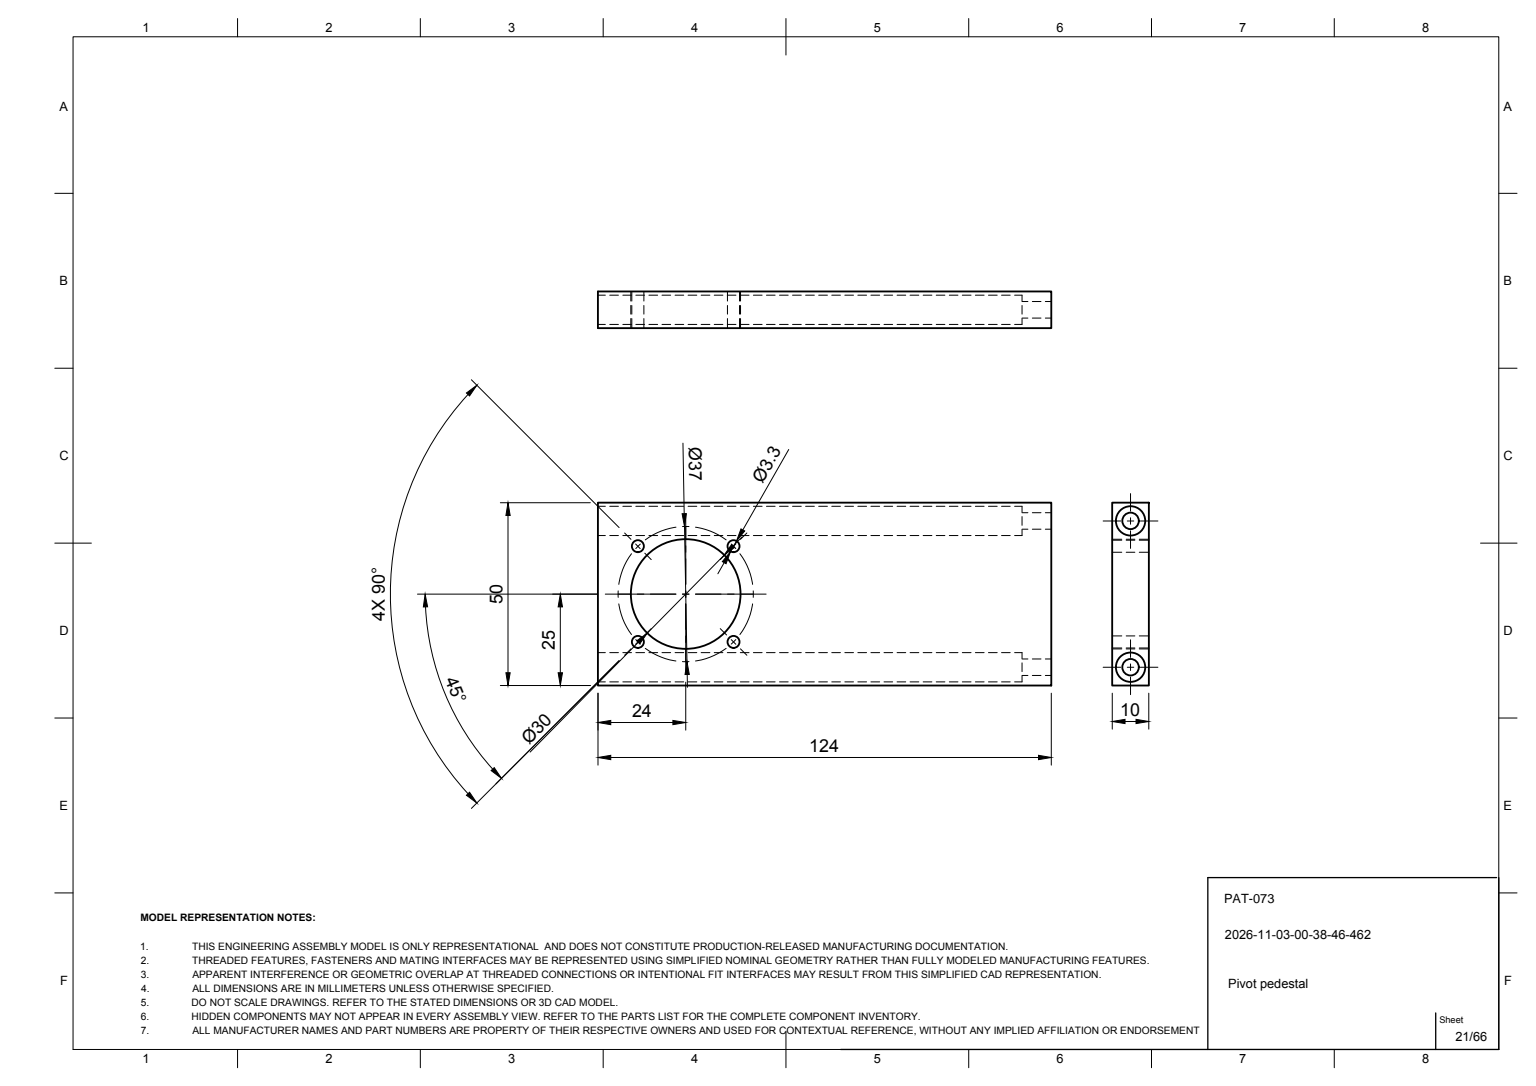
ISO-10303-21;
HEADER;
/* Generated by software containing ST-Developer
 * from STEP Tools, Inc. (www.steptools.com) 
 */

FILE_DESCRIPTION(
/* description */ ('Manual piston pump'),
/* implementation_level */ '2;1');

FILE_NAME(
/* name */ 'Pivot pedestal.step',
/* time_stamp */ '2026-11-02T16:54:23-08:00',
/* author */ (''),
/* organization */ (''),
/* preprocessor_version */ 'ST-DEVELOPER v20.2',
/* originating_system */ 'Autodesk Translation Framework v15.17.0.0',
/* authorisation */ '');

FILE_SCHEMA (('AUTOMOTIVE_DESIGN { 1 0 10303 214 3 1 1 }'));
ENDSEC;

DATA;
#10=MECHANICAL_DESIGN_GEOMETRIC_PRESENTATION_REPRESENTATION('',(#707),#19043);
#581=SHAPE_REPRESENTATION_RELATIONSHIP('SRR','None',#19327,#644);
#644=ADVANCED_BREP_SHAPE_REPRESENTATION('',(#778),#18994);
#707=STYLED_ITEM('',(#19661),#778);
#778=MANIFOLD_SOLID_BREP('Body1',#9492);
#901=FACE_BOUND('',#2123,.T.);
#902=FACE_BOUND('',#2127,.T.);
#903=FACE_BOUND('',#2131,.T.);
#904=FACE_BOUND('',#2132,.T.);
#905=FACE_BOUND('',#2135,.T.);
#906=FACE_BOUND('',#2136,.T.);
#907=FACE_BOUND('',#2139,.T.);
#908=FACE_BOUND('',#2140,.T.);
#909=FACE_BOUND('',#2141,.T.);
#910=FACE_BOUND('',#2142,.T.);
#911=FACE_BOUND('',#2143,.T.);
#912=FACE_BOUND('',#2145,.T.);
#913=FACE_BOUND('',#2146,.T.);
#914=FACE_BOUND('',#2147,.T.);
#915=FACE_BOUND('',#2148,.T.);
#916=FACE_BOUND('',#2149,.T.);
#1155=CYLINDRICAL_SURFACE('',#10580,0.164999999999999);
#1156=CYLINDRICAL_SURFACE('',#10583,0.164999999999999);
#1157=CYLINDRICAL_SURFACE('',#10586,0.164999999999999);
#1158=CYLINDRICAL_SURFACE('',#10589,0.164999999999999);
#1159=CYLINDRICAL_SURFACE('',#10592,0.4);
#1160=CYLINDRICAL_SURFACE('',#10597,0.225);
#1161=CYLINDRICAL_SURFACE('',#10599,0.4);
#1162=CYLINDRICAL_SURFACE('',#10604,0.225);
#1163=CYLINDRICAL_SURFACE('',#10606,1.5);
#1468=FACE_OUTER_BOUND('',#2117,.T.);
#1469=FACE_OUTER_BOUND('',#2118,.T.);
#1470=FACE_OUTER_BOUND('',#2119,.T.);
#1471=FACE_OUTER_BOUND('',#2120,.T.);
#1472=FACE_OUTER_BOUND('',#2121,.T.);
#1473=FACE_OUTER_BOUND('',#2122,.T.);
#1474=FACE_OUTER_BOUND('',#2124,.T.);
#1475=FACE_OUTER_BOUND('',#2125,.T.);
#1476=FACE_OUTER_BOUND('',#2126,.T.);
#1477=FACE_OUTER_BOUND('',#2128,.T.);
#1478=FACE_OUTER_BOUND('',#2129,.T.);
#1479=FACE_OUTER_BOUND('',#2130,.T.);
#1480=FACE_OUTER_BOUND('',#2133,.T.);
#1481=FACE_OUTER_BOUND('',#2134,.T.);
#1482=FACE_OUTER_BOUND('',#2137,.T.);
#1483=FACE_OUTER_BOUND('',#2138,.T.);
#1484=FACE_OUTER_BOUND('',#2144,.T.);
#2117=EDGE_LOOP('',(#6985,#6986,#6987,#6988));
#2118=EDGE_LOOP('',(#6989,#6990,#6991,#6992));
#2119=EDGE_LOOP('',(#6993,#6994,#6995,#6996));
#2120=EDGE_LOOP('',(#6997,#6998,#6999,#7000));
#2121=EDGE_LOOP('',(#7001,#7002,#7003,#7004));
#2122=EDGE_LOOP('',(#7005));
#2123=EDGE_LOOP('',(#7006));
#2124=EDGE_LOOP('',(#7007,#7008,#7009,#7010));
#2125=EDGE_LOOP('',(#7011,#7012,#7013,#7014));
#2126=EDGE_LOOP('',(#7015));
#2127=EDGE_LOOP('',(#7016));
#2128=EDGE_LOOP('',(#7017,#7018,#7019,#7020));
#2129=EDGE_LOOP('',(#7021,#7022,#7023,#7024));
#2130=EDGE_LOOP('',(#7025,#7026,#7027,#7028));
#2131=EDGE_LOOP('',(#7029));
#2132=EDGE_LOOP('',(#7030));
#2133=EDGE_LOOP('',(#7031,#7032,#7033,#7034));
#2134=EDGE_LOOP('',(#7035,#7036,#7037,#7038));
#2135=EDGE_LOOP('',(#7039));
#2136=EDGE_LOOP('',(#7040));
#2137=EDGE_LOOP('',(#7041,#7042,#7043,#7044));
#2138=EDGE_LOOP('',(#7045,#7046,#7047,#7048));
#2139=EDGE_LOOP('',(#7049));
#2140=EDGE_LOOP('',(#7050));
#2141=EDGE_LOOP('',(#7051));
#2142=EDGE_LOOP('',(#7052));
#2143=EDGE_LOOP('',(#7053));
#2144=EDGE_LOOP('',(#7054,#7055,#7056,#7057));
#2145=EDGE_LOOP('',(#7058));
#2146=EDGE_LOOP('',(#7059));
#2147=EDGE_LOOP('',(#7060));
#2148=EDGE_LOOP('',(#7061));
#2149=EDGE_LOOP('',(#7062));
#2802=CIRCLE('',#10581,0.164999999999999);
#2803=CIRCLE('',#10582,0.164999999999999);
#2804=CIRCLE('',#10584,0.164999999999999);
#2805=CIRCLE('',#10585,0.164999999999999);
#2806=CIRCLE('',#10587,0.164999999999999);
#2807=CIRCLE('',#10588,0.164999999999999);
#2808=CIRCLE('',#10590,0.164999999999999);
#2809=CIRCLE('',#10591,0.164999999999999);
#2810=CIRCLE('',#10593,0.4);
#2811=CIRCLE('',#10594,0.4);
#2812=CIRCLE('',#10596,0.225);
#2813=CIRCLE('',#10598,0.225);
#2814=CIRCLE('',#10600,0.4);
#2815=CIRCLE('',#10601,0.4);
#2816=CIRCLE('',#10603,0.225);
#2817=CIRCLE('',#10605,0.225);
#2818=CIRCLE('',#10607,1.5);
#2819=CIRCLE('',#10608,1.5);
#3349=LINE('',#15470,#3953);
#3350=LINE('',#15476,#3954);
#3351=LINE('',#15482,#3955);
#3352=LINE('',#15488,#3956);
#3353=LINE('',#15494,#3957);
#3354=LINE('',#15502,#3958);
#3355=LINE('',#15507,#3959);
#3356=LINE('',#15515,#3960);
#3357=LINE('',#15520,#3961);
#3358=LINE('',#15525,#3962);
#3359=LINE('',#15527,#3963);
#3360=LINE('',#15529,#3964);
#3361=LINE('',#15530,#3965);
#3362=LINE('',#15533,#3966);
#3363=LINE('',#15535,#3967);
#3364=LINE('',#15536,#3968);
#3365=LINE('',#15539,#3969);
#3366=LINE('',#15541,#3970);
#3367=LINE('',#15542,#3971);
#3368=LINE('',#15544,#3972);
#3369=LINE('',#15545,#3973);
#3953=VECTOR('',#12375,0.164999999999999);
#3954=VECTOR('',#12382,0.164999999999999);
#3955=VECTOR('',#12389,0.164999999999999);
#3956=VECTOR('',#12396,0.164999999999999);
#3957=VECTOR('',#12403,0.4);
#3958=VECTOR('',#12414,0.225);
#3959=VECTOR('',#12419,0.4);
#3960=VECTOR('',#12430,0.225);
#3961=VECTOR('',#12435,1.5);
#3962=VECTOR('',#12440,1.);
#3963=VECTOR('',#12441,1.);
#3964=VECTOR('',#12442,1.);
#3965=VECTOR('',#12443,1.);
#3966=VECTOR('',#12446,1.);
#3967=VECTOR('',#12447,1.);
#3968=VECTOR('',#12448,1.);
#3969=VECTOR('',#12451,1.);
#3970=VECTOR('',#12452,1.);
#3971=VECTOR('',#12453,1.);
#3972=VECTOR('',#12456,1.);
#3973=VECTOR('',#12457,1.);
#4589=VERTEX_POINT('',#15467);
#4590=VERTEX_POINT('',#15469);
#4591=VERTEX_POINT('',#15473);
#4592=VERTEX_POINT('',#15475);
#4593=VERTEX_POINT('',#15479);
#4594=VERTEX_POINT('',#15481);
#4595=VERTEX_POINT('',#15485);
#4596=VERTEX_POINT('',#15487);
#4597=VERTEX_POINT('',#15491);
#4598=VERTEX_POINT('',#15493);
#4599=VERTEX_POINT('',#15497);
#4600=VERTEX_POINT('',#15500);
#4601=VERTEX_POINT('',#15504);
#4602=VERTEX_POINT('',#15506);
#4603=VERTEX_POINT('',#15510);
#4604=VERTEX_POINT('',#15513);
#4605=VERTEX_POINT('',#15517);
#4606=VERTEX_POINT('',#15519);
#4607=VERTEX_POINT('',#15523);
#4608=VERTEX_POINT('',#15524);
#4609=VERTEX_POINT('',#15526);
#4610=VERTEX_POINT('',#15528);
#4611=VERTEX_POINT('',#15532);
#4612=VERTEX_POINT('',#15534);
#4613=VERTEX_POINT('',#15538);
#4614=VERTEX_POINT('',#15540);
#5479=EDGE_CURVE('',#4589,#4589,#2802,.T.);
#5480=EDGE_CURVE('',#4589,#4590,#3349,.T.);
#5481=EDGE_CURVE('',#4590,#4590,#2803,.T.);
#5482=EDGE_CURVE('',#4591,#4591,#2804,.T.);
#5483=EDGE_CURVE('',#4591,#4592,#3350,.T.);
#5484=EDGE_CURVE('',#4592,#4592,#2805,.T.);
#5485=EDGE_CURVE('',#4593,#4593,#2806,.T.);
#5486=EDGE_CURVE('',#4593,#4594,#3351,.T.);
#5487=EDGE_CURVE('',#4594,#4594,#2807,.T.);
#5488=EDGE_CURVE('',#4595,#4595,#2808,.T.);
#5489=EDGE_CURVE('',#4595,#4596,#3352,.T.);
#5490=EDGE_CURVE('',#4596,#4596,#2809,.T.);
#5491=EDGE_CURVE('',#4597,#4597,#2810,.T.);
#5492=EDGE_CURVE('',#4597,#4598,#3353,.T.);
#5493=EDGE_CURVE('',#4598,#4598,#2811,.T.);
#5494=EDGE_CURVE('',#4599,#4599,#2812,.T.);
#5495=EDGE_CURVE('',#4600,#4600,#2813,.T.);
#5496=EDGE_CURVE('',#4600,#4599,#3354,.T.);
#5497=EDGE_CURVE('',#4601,#4601,#2814,.T.);
#5498=EDGE_CURVE('',#4601,#4602,#3355,.T.);
#5499=EDGE_CURVE('',#4602,#4602,#2815,.T.);
#5500=EDGE_CURVE('',#4603,#4603,#2816,.T.);
#5501=EDGE_CURVE('',#4604,#4604,#2817,.T.);
#5502=EDGE_CURVE('',#4604,#4603,#3356,.T.);
#5503=EDGE_CURVE('',#4605,#4605,#2818,.T.);
#5504=EDGE_CURVE('',#4605,#4606,#3357,.T.);
#5505=EDGE_CURVE('',#4606,#4606,#2819,.T.);
#5506=EDGE_CURVE('',#4607,#4608,#3358,.T.);
#5507=EDGE_CURVE('',#4608,#4609,#3359,.T.);
#5508=EDGE_CURVE('',#4610,#4609,#3360,.T.);
#5509=EDGE_CURVE('',#4607,#4610,#3361,.T.);
#5510=EDGE_CURVE('',#4611,#4607,#3362,.T.);
#5511=EDGE_CURVE('',#4612,#4610,#3363,.T.);
#5512=EDGE_CURVE('',#4611,#4612,#3364,.T.);
#5513=EDGE_CURVE('',#4613,#4611,#3365,.T.);
#5514=EDGE_CURVE('',#4614,#4612,#3366,.T.);
#5515=EDGE_CURVE('',#4613,#4614,#3367,.T.);
#5516=EDGE_CURVE('',#4608,#4613,#3368,.T.);
#5517=EDGE_CURVE('',#4609,#4614,#3369,.T.);
#6985=ORIENTED_EDGE('',*,*,#5479,.F.);
#6986=ORIENTED_EDGE('',*,*,#5480,.T.);
#6987=ORIENTED_EDGE('',*,*,#5481,.F.);
#6988=ORIENTED_EDGE('',*,*,#5480,.F.);
#6989=ORIENTED_EDGE('',*,*,#5482,.F.);
#6990=ORIENTED_EDGE('',*,*,#5483,.T.);
#6991=ORIENTED_EDGE('',*,*,#5484,.F.);
#6992=ORIENTED_EDGE('',*,*,#5483,.F.);
#6993=ORIENTED_EDGE('',*,*,#5485,.F.);
#6994=ORIENTED_EDGE('',*,*,#5486,.T.);
#6995=ORIENTED_EDGE('',*,*,#5487,.F.);
#6996=ORIENTED_EDGE('',*,*,#5486,.F.);
#6997=ORIENTED_EDGE('',*,*,#5488,.F.);
#6998=ORIENTED_EDGE('',*,*,#5489,.T.);
#6999=ORIENTED_EDGE('',*,*,#5490,.F.);
#7000=ORIENTED_EDGE('',*,*,#5489,.F.);
#7001=ORIENTED_EDGE('',*,*,#5491,.F.);
#7002=ORIENTED_EDGE('',*,*,#5492,.T.);
#7003=ORIENTED_EDGE('',*,*,#5493,.F.);
#7004=ORIENTED_EDGE('',*,*,#5492,.F.);
#7005=ORIENTED_EDGE('',*,*,#5491,.T.);
#7006=ORIENTED_EDGE('',*,*,#5494,.F.);
#7007=ORIENTED_EDGE('',*,*,#5495,.F.);
#7008=ORIENTED_EDGE('',*,*,#5496,.T.);
#7009=ORIENTED_EDGE('',*,*,#5494,.T.);
#7010=ORIENTED_EDGE('',*,*,#5496,.F.);
#7011=ORIENTED_EDGE('',*,*,#5497,.F.);
#7012=ORIENTED_EDGE('',*,*,#5498,.T.);
#7013=ORIENTED_EDGE('',*,*,#5499,.F.);
#7014=ORIENTED_EDGE('',*,*,#5498,.F.);
#7015=ORIENTED_EDGE('',*,*,#5497,.T.);
#7016=ORIENTED_EDGE('',*,*,#5500,.F.);
#7017=ORIENTED_EDGE('',*,*,#5501,.F.);
#7018=ORIENTED_EDGE('',*,*,#5502,.T.);
#7019=ORIENTED_EDGE('',*,*,#5500,.T.);
#7020=ORIENTED_EDGE('',*,*,#5502,.F.);
#7021=ORIENTED_EDGE('',*,*,#5503,.F.);
#7022=ORIENTED_EDGE('',*,*,#5504,.T.);
#7023=ORIENTED_EDGE('',*,*,#5505,.F.);
#7024=ORIENTED_EDGE('',*,*,#5504,.F.);
#7025=ORIENTED_EDGE('',*,*,#5506,.T.);
#7026=ORIENTED_EDGE('',*,*,#5507,.T.);
#7027=ORIENTED_EDGE('',*,*,#5508,.F.);
#7028=ORIENTED_EDGE('',*,*,#5509,.F.);
#7029=ORIENTED_EDGE('',*,*,#5493,.T.);
#7030=ORIENTED_EDGE('',*,*,#5499,.T.);
#7031=ORIENTED_EDGE('',*,*,#5510,.T.);
#7032=ORIENTED_EDGE('',*,*,#5509,.T.);
#7033=ORIENTED_EDGE('',*,*,#5511,.F.);
#7034=ORIENTED_EDGE('',*,*,#5512,.F.);
#7035=ORIENTED_EDGE('',*,*,#5513,.T.);
#7036=ORIENTED_EDGE('',*,*,#5512,.T.);
#7037=ORIENTED_EDGE('',*,*,#5514,.F.);
#7038=ORIENTED_EDGE('',*,*,#5515,.F.);
#7039=ORIENTED_EDGE('',*,*,#5495,.T.);
#7040=ORIENTED_EDGE('',*,*,#5501,.T.);
#7041=ORIENTED_EDGE('',*,*,#5516,.T.);
#7042=ORIENTED_EDGE('',*,*,#5515,.T.);
#7043=ORIENTED_EDGE('',*,*,#5517,.F.);
#7044=ORIENTED_EDGE('',*,*,#5507,.F.);
#7045=ORIENTED_EDGE('',*,*,#5517,.T.);
#7046=ORIENTED_EDGE('',*,*,#5514,.T.);
#7047=ORIENTED_EDGE('',*,*,#5511,.T.);
#7048=ORIENTED_EDGE('',*,*,#5508,.T.);
#7049=ORIENTED_EDGE('',*,*,#5505,.T.);
#7050=ORIENTED_EDGE('',*,*,#5490,.T.);
#7051=ORIENTED_EDGE('',*,*,#5487,.T.);
#7052=ORIENTED_EDGE('',*,*,#5484,.T.);
#7053=ORIENTED_EDGE('',*,*,#5481,.T.);
#7054=ORIENTED_EDGE('',*,*,#5516,.F.);
#7055=ORIENTED_EDGE('',*,*,#5506,.F.);
#7056=ORIENTED_EDGE('',*,*,#5510,.F.);
#7057=ORIENTED_EDGE('',*,*,#5513,.F.);
#7058=ORIENTED_EDGE('',*,*,#5503,.T.);
#7059=ORIENTED_EDGE('',*,*,#5488,.T.);
#7060=ORIENTED_EDGE('',*,*,#5485,.T.);
#7061=ORIENTED_EDGE('',*,*,#5482,.T.);
#7062=ORIENTED_EDGE('',*,*,#5479,.T.);
#8677=PLANE('',#10595);
#8678=PLANE('',#10602);
#8679=PLANE('',#10609);
#8680=PLANE('',#10610);
#8681=PLANE('',#10611);
#8682=PLANE('',#10612);
#8683=PLANE('',#10613);
#8684=PLANE('',#10614);
#9073=ADVANCED_FACE('',(#1468),#1155,.F.);
#9074=ADVANCED_FACE('',(#1469),#1156,.F.);
#9075=ADVANCED_FACE('',(#1470),#1157,.F.);
#9076=ADVANCED_FACE('',(#1471),#1158,.F.);
#9077=ADVANCED_FACE('',(#1472),#1159,.F.);
#9078=ADVANCED_FACE('',(#1473,#901),#8677,.T.);
#9079=ADVANCED_FACE('',(#1474),#1160,.F.);
#9080=ADVANCED_FACE('',(#1475),#1161,.F.);
#9081=ADVANCED_FACE('',(#1476,#902),#8678,.T.);
#9082=ADVANCED_FACE('',(#1477),#1162,.F.);
#9083=ADVANCED_FACE('',(#1478),#1163,.F.);
#9084=ADVANCED_FACE('',(#1479,#903,#904),#8679,.T.);
#9085=ADVANCED_FACE('',(#1480),#8680,.T.);
#9086=ADVANCED_FACE('',(#1481,#905,#906),#8681,.T.);
#9087=ADVANCED_FACE('',(#1482),#8682,.T.);
#9088=ADVANCED_FACE('',(#1483,#907,#908,#909,#910,#911),#8683,.T.);
#9089=ADVANCED_FACE('',(#1484,#912,#913,#914,#915,#916),#8684,.F.);
#9492=CLOSED_SHELL('',(#9073,#9074,#9075,#9076,#9077,#9078,#9079,#9080,
#9081,#9082,#9083,#9084,#9085,#9086,#9087,#9088,#9089));
#10579=AXIS2_PLACEMENT_3D('',#15465,#12369,#12370);
#10580=AXIS2_PLACEMENT_3D('',#15466,#12371,#12372);
#10581=AXIS2_PLACEMENT_3D('',#15468,#12373,#12374);
#10582=AXIS2_PLACEMENT_3D('',#15471,#12376,#12377);
#10583=AXIS2_PLACEMENT_3D('',#15472,#12378,#12379);
#10584=AXIS2_PLACEMENT_3D('',#15474,#12380,#12381);
#10585=AXIS2_PLACEMENT_3D('',#15477,#12383,#12384);
#10586=AXIS2_PLACEMENT_3D('',#15478,#12385,#12386);
#10587=AXIS2_PLACEMENT_3D('',#15480,#12387,#12388);
#10588=AXIS2_PLACEMENT_3D('',#15483,#12390,#12391);
#10589=AXIS2_PLACEMENT_3D('',#15484,#12392,#12393);
#10590=AXIS2_PLACEMENT_3D('',#15486,#12394,#12395);
#10591=AXIS2_PLACEMENT_3D('',#15489,#12397,#12398);
#10592=AXIS2_PLACEMENT_3D('',#15490,#12399,#12400);
#10593=AXIS2_PLACEMENT_3D('',#15492,#12401,#12402);
#10594=AXIS2_PLACEMENT_3D('',#15495,#12404,#12405);
#10595=AXIS2_PLACEMENT_3D('',#15496,#12406,#12407);
#10596=AXIS2_PLACEMENT_3D('',#15498,#12408,#12409);
#10597=AXIS2_PLACEMENT_3D('',#15499,#12410,#12411);
#10598=AXIS2_PLACEMENT_3D('',#15501,#12412,#12413);
#10599=AXIS2_PLACEMENT_3D('',#15503,#12415,#12416);
#10600=AXIS2_PLACEMENT_3D('',#15505,#12417,#12418);
#10601=AXIS2_PLACEMENT_3D('',#15508,#12420,#12421);
#10602=AXIS2_PLACEMENT_3D('',#15509,#12422,#12423);
#10603=AXIS2_PLACEMENT_3D('',#15511,#12424,#12425);
#10604=AXIS2_PLACEMENT_3D('',#15512,#12426,#12427);
#10605=AXIS2_PLACEMENT_3D('',#15514,#12428,#12429);
#10606=AXIS2_PLACEMENT_3D('',#15516,#12431,#12432);
#10607=AXIS2_PLACEMENT_3D('',#15518,#12433,#12434);
#10608=AXIS2_PLACEMENT_3D('',#15521,#12436,#12437);
#10609=AXIS2_PLACEMENT_3D('',#15522,#12438,#12439);
#10610=AXIS2_PLACEMENT_3D('',#15531,#12444,#12445);
#10611=AXIS2_PLACEMENT_3D('',#15537,#12449,#12450);
#10612=AXIS2_PLACEMENT_3D('',#15543,#12454,#12455);
#10613=AXIS2_PLACEMENT_3D('',#15546,#12458,#12459);
#10614=AXIS2_PLACEMENT_3D('',#15547,#12460,#12461);
#12369=DIRECTION('axis',(0.,0.,1.));
#12370=DIRECTION('refdir',(1.,0.,0.));
#12371=DIRECTION('center_axis',(1.,0.,0.));
#12372=DIRECTION('ref_axis',(0.,0.,-1.));
#12373=DIRECTION('center_axis',(1.,0.,0.));
#12374=DIRECTION('ref_axis',(0.,0.,-1.));
#12375=DIRECTION('',(1.,0.,0.));
#12376=DIRECTION('center_axis',(-1.,0.,0.));
#12377=DIRECTION('ref_axis',(0.,0.,-1.));
#12378=DIRECTION('center_axis',(1.,0.,0.));
#12379=DIRECTION('ref_axis',(0.,0.,-1.));
#12380=DIRECTION('center_axis',(1.,0.,0.));
#12381=DIRECTION('ref_axis',(0.,0.,-1.));
#12382=DIRECTION('',(1.,0.,0.));
#12383=DIRECTION('center_axis',(-1.,0.,0.));
#12384=DIRECTION('ref_axis',(0.,0.,-1.));
#12385=DIRECTION('center_axis',(1.,0.,0.));
#12386=DIRECTION('ref_axis',(0.,0.,-1.));
#12387=DIRECTION('center_axis',(1.,0.,0.));
#12388=DIRECTION('ref_axis',(0.,0.,-1.));
#12389=DIRECTION('',(1.,0.,0.));
#12390=DIRECTION('center_axis',(-1.,0.,0.));
#12391=DIRECTION('ref_axis',(0.,0.,-1.));
#12392=DIRECTION('center_axis',(1.,0.,0.));
#12393=DIRECTION('ref_axis',(0.,0.,-1.));
#12394=DIRECTION('center_axis',(1.,0.,0.));
#12395=DIRECTION('ref_axis',(0.,0.,-1.));
#12396=DIRECTION('',(1.,0.,0.));
#12397=DIRECTION('center_axis',(-1.,0.,0.));
#12398=DIRECTION('ref_axis',(0.,0.,-1.));
#12399=DIRECTION('center_axis',(0.,0.,1.));
#12400=DIRECTION('ref_axis',(1.,0.,0.));
#12401=DIRECTION('center_axis',(0.,0.,1.));
#12402=DIRECTION('ref_axis',(1.,0.,0.));
#12403=DIRECTION('',(0.,0.,1.));
#12404=DIRECTION('center_axis',(0.,0.,-1.));
#12405=DIRECTION('ref_axis',(1.,0.,0.));
#12406=DIRECTION('center_axis',(0.,0.,1.));
#12407=DIRECTION('ref_axis',(1.,0.,0.));
#12408=DIRECTION('center_axis',(0.,0.,1.));
#12409=DIRECTION('ref_axis',(1.,0.,0.));
#12410=DIRECTION('center_axis',(0.,0.,1.));
#12411=DIRECTION('ref_axis',(1.,0.,0.));
#12412=DIRECTION('center_axis',(0.,0.,1.));
#12413=DIRECTION('ref_axis',(1.,0.,0.));
#12414=DIRECTION('',(0.,0.,1.));
#12415=DIRECTION('center_axis',(0.,0.,1.));
#12416=DIRECTION('ref_axis',(1.,0.,0.));
#12417=DIRECTION('center_axis',(0.,0.,1.));
#12418=DIRECTION('ref_axis',(1.,0.,0.));
#12419=DIRECTION('',(0.,0.,1.));
#12420=DIRECTION('center_axis',(0.,0.,-1.));
#12421=DIRECTION('ref_axis',(1.,0.,0.));
#12422=DIRECTION('center_axis',(0.,0.,1.));
#12423=DIRECTION('ref_axis',(1.,0.,0.));
#12424=DIRECTION('center_axis',(0.,0.,1.));
#12425=DIRECTION('ref_axis',(1.,0.,0.));
#12426=DIRECTION('center_axis',(0.,0.,1.));
#12427=DIRECTION('ref_axis',(1.,0.,0.));
#12428=DIRECTION('center_axis',(0.,0.,1.));
#12429=DIRECTION('ref_axis',(1.,0.,0.));
#12430=DIRECTION('',(0.,0.,1.));
#12431=DIRECTION('center_axis',(1.,0.,0.));
#12432=DIRECTION('ref_axis',(0.,0.,-1.));
#12433=DIRECTION('center_axis',(1.,0.,0.));
#12434=DIRECTION('ref_axis',(0.,0.,-1.));
#12435=DIRECTION('',(1.,0.,0.));
#12436=DIRECTION('center_axis',(-1.,0.,0.));
#12437=DIRECTION('ref_axis',(0.,0.,-1.));
#12438=DIRECTION('center_axis',(0.,0.,1.));
#12439=DIRECTION('ref_axis',(0.,-1.,0.));
#12440=DIRECTION('',(0.,-1.,0.));
#12441=DIRECTION('',(1.,0.,0.));
#12442=DIRECTION('',(0.,-1.,0.));
#12443=DIRECTION('',(1.,0.,0.));
#12444=DIRECTION('center_axis',(0.,1.,0.));
#12445=DIRECTION('ref_axis',(0.,0.,1.));
#12446=DIRECTION('',(0.,0.,1.));
#12447=DIRECTION('',(0.,0.,1.));
#12448=DIRECTION('',(1.,0.,0.));
#12449=DIRECTION('center_axis',(0.,0.,-1.));
#12450=DIRECTION('ref_axis',(0.,1.,0.));
#12451=DIRECTION('',(0.,1.,0.));
#12452=DIRECTION('',(0.,1.,0.));
#12453=DIRECTION('',(1.,0.,0.));
#12454=DIRECTION('center_axis',(0.,-1.,0.));
#12455=DIRECTION('ref_axis',(0.,0.,-1.));
#12456=DIRECTION('',(0.,0.,-1.));
#12457=DIRECTION('',(0.,0.,-1.));
#12458=DIRECTION('center_axis',(1.,0.,0.));
#12459=DIRECTION('ref_axis',(0.,0.,-1.));
#12460=DIRECTION('center_axis',(1.,0.,0.));
#12461=DIRECTION('ref_axis',(0.,0.,-1.));
#15465=CARTESIAN_POINT('',(0.,0.,0.));
#15466=CARTESIAN_POINT('Origin',(-3.1,-5.30814754519511,8.69185245480489));
#15467=CARTESIAN_POINT('',(-3.,-5.30814754519511,8.85685245480489));
#15468=CARTESIAN_POINT('Origin',(-3.,-5.30814754519511,8.69185245480489));
#15469=CARTESIAN_POINT('',(-2.,-5.30814754519511,8.85685245480489));
#15470=CARTESIAN_POINT('',(-3.1,-5.30814754519511,8.85685245480489));
#15471=CARTESIAN_POINT('Origin',(-2.,-5.30814754519511,8.69185245480489));
#15472=CARTESIAN_POINT('Origin',(-3.1,-5.30814754519511,11.3081475451951));
#15473=CARTESIAN_POINT('',(-3.,-5.30814754519511,11.4731475451951));
#15474=CARTESIAN_POINT('Origin',(-3.,-5.30814754519511,11.3081475451951));
#15475=CARTESIAN_POINT('',(-2.,-5.30814754519511,11.4731475451951));
#15476=CARTESIAN_POINT('',(-3.1,-5.30814754519511,11.4731475451951));
#15477=CARTESIAN_POINT('Origin',(-2.,-5.30814754519511,11.3081475451951));
#15478=CARTESIAN_POINT('Origin',(-3.1,-2.69185245480489,11.3081475451951));
#15479=CARTESIAN_POINT('',(-3.,-2.69185245480489,11.4731475451951));
#15480=CARTESIAN_POINT('Origin',(-3.,-2.69185245480489,11.3081475451951));
#15481=CARTESIAN_POINT('',(-2.,-2.69185245480489,11.4731475451951));
#15482=CARTESIAN_POINT('',(-3.1,-2.69185245480489,11.4731475451951));
#15483=CARTESIAN_POINT('Origin',(-2.,-2.69185245480489,11.3081475451951));
#15484=CARTESIAN_POINT('Origin',(-3.1,-2.69185245480489,8.69185245480489));
#15485=CARTESIAN_POINT('',(-3.,-2.69185245480489,8.85685245480489));
#15486=CARTESIAN_POINT('Origin',(-3.,-2.69185245480489,8.69185245480489));
#15487=CARTESIAN_POINT('',(-2.,-2.69185245480489,8.85685245480489));
#15488=CARTESIAN_POINT('',(-3.1,-2.69185245480489,8.85685245480489));
#15489=CARTESIAN_POINT('Origin',(-2.,-2.69185245480489,8.69185245480489));
#15490=CARTESIAN_POINT('Origin',(-2.5,-2.,0.8));
#15491=CARTESIAN_POINT('',(-2.9,-2.,0.8));
#15492=CARTESIAN_POINT('Origin',(-2.5,-2.,0.8));
#15493=CARTESIAN_POINT('',(-2.9,-2.,12.4));
#15494=CARTESIAN_POINT('',(-2.9,-2.,0.8));
#15495=CARTESIAN_POINT('Origin',(-2.5,-2.,12.4));
#15496=CARTESIAN_POINT('Origin',(-2.5,-2.,0.8));
#15497=CARTESIAN_POINT('',(-2.725,-2.,0.8));
#15498=CARTESIAN_POINT('Origin',(-2.5,-2.,0.8));
#15499=CARTESIAN_POINT('Origin',(-2.5,-2.,-0.1));
#15500=CARTESIAN_POINT('',(-2.725,-2.,0.));
#15501=CARTESIAN_POINT('Origin',(-2.5,-2.,0.));
#15502=CARTESIAN_POINT('',(-2.725,-2.,-0.1));
#15503=CARTESIAN_POINT('Origin',(-2.5,-6.,0.8));
#15504=CARTESIAN_POINT('',(-2.9,-6.,0.8));
#15505=CARTESIAN_POINT('Origin',(-2.5,-6.,0.8));
#15506=CARTESIAN_POINT('',(-2.9,-6.,12.4));
#15507=CARTESIAN_POINT('',(-2.9,-6.,0.8));
#15508=CARTESIAN_POINT('Origin',(-2.5,-6.,12.4));
#15509=CARTESIAN_POINT('Origin',(-2.5,-6.,0.8));
#15510=CARTESIAN_POINT('',(-2.725,-6.,0.8));
#15511=CARTESIAN_POINT('Origin',(-2.5,-6.,0.8));
#15512=CARTESIAN_POINT('Origin',(-2.5,-6.,-0.1));
#15513=CARTESIAN_POINT('',(-2.725,-6.,0.));
#15514=CARTESIAN_POINT('Origin',(-2.5,-6.,0.));
#15515=CARTESIAN_POINT('',(-2.725,-6.,-0.1));
#15516=CARTESIAN_POINT('Origin',(-3.1,-4.,10.));
#15517=CARTESIAN_POINT('',(-3.,-4.,11.5));
#15518=CARTESIAN_POINT('Origin',(-3.,-4.,10.));
#15519=CARTESIAN_POINT('',(-2.,-4.,11.5));
#15520=CARTESIAN_POINT('',(-3.1,-4.,11.5));
#15521=CARTESIAN_POINT('Origin',(-2.,-4.,10.));
#15522=CARTESIAN_POINT('Origin',(-3.,-1.5,12.4));
#15523=CARTESIAN_POINT('',(-3.,-1.5,12.4));
#15524=CARTESIAN_POINT('',(-3.,-6.5,12.4));
#15525=CARTESIAN_POINT('',(-3.,-1.5,12.4));
#15526=CARTESIAN_POINT('',(-2.,-6.5,12.4));
#15527=CARTESIAN_POINT('',(-3.,-6.5,12.4));
#15528=CARTESIAN_POINT('',(-2.,-1.5,12.4));
#15529=CARTESIAN_POINT('',(-2.,-1.5,12.4));
#15530=CARTESIAN_POINT('',(-3.,-1.5,12.4));
#15531=CARTESIAN_POINT('Origin',(-3.,-1.5,0.));
#15532=CARTESIAN_POINT('',(-3.,-1.5,0.));
#15533=CARTESIAN_POINT('',(-3.,-1.5,0.));
#15534=CARTESIAN_POINT('',(-2.,-1.5,0.));
#15535=CARTESIAN_POINT('',(-2.,-1.5,0.));
#15536=CARTESIAN_POINT('',(-3.,-1.5,0.));
#15537=CARTESIAN_POINT('Origin',(-3.,-6.5,0.));
#15538=CARTESIAN_POINT('',(-3.,-6.5,0.));
#15539=CARTESIAN_POINT('',(-3.,-6.5,0.));
#15540=CARTESIAN_POINT('',(-2.,-6.5,0.));
#15541=CARTESIAN_POINT('',(-2.,-6.5,0.));
#15542=CARTESIAN_POINT('',(-3.,-6.5,0.));
#15543=CARTESIAN_POINT('Origin',(-3.,-6.5,12.4));
#15544=CARTESIAN_POINT('',(-3.,-6.5,12.4));
#15545=CARTESIAN_POINT('',(-2.,-6.5,12.4));
#15546=CARTESIAN_POINT('Origin',(-2.,-4.,6.2));
#15547=CARTESIAN_POINT('Origin',(-3.,-4.,6.2));
#18923=UNCERTAINTY_MEASURE_WITH_UNIT(LENGTH_MEASURE(0.001),#19044,
'DISTANCE_ACCURACY_VALUE',
'Maximum model space distance between geometric entities at asserted c
onnectivities');
#18972=UNCERTAINTY_MEASURE_WITH_UNIT(LENGTH_MEASURE(0.001),#19044,
'DISTANCE_ACCURACY_VALUE',
'Maximum model space distance between geometric entities at asserted c
onnectivities');
#18994=(
GEOMETRIC_REPRESENTATION_CONTEXT(3)
GLOBAL_UNCERTAINTY_ASSIGNED_CONTEXT((#18923))
GLOBAL_UNIT_ASSIGNED_CONTEXT((#19044,#19046,#19047))
REPRESENTATION_CONTEXT('','3D')
);
#19043=(
GEOMETRIC_REPRESENTATION_CONTEXT(3)
GLOBAL_UNCERTAINTY_ASSIGNED_CONTEXT((#18972))
GLOBAL_UNIT_ASSIGNED_CONTEXT((#19044,#19046,#19047))
REPRESENTATION_CONTEXT('','3D')
);
#19044=(
LENGTH_UNIT()
NAMED_UNIT(*)
SI_UNIT(.CENTI.,.METRE.)
);
#19046=(
NAMED_UNIT(*)
PLANE_ANGLE_UNIT()
SI_UNIT($,.RADIAN.)
);
#19047=(
NAMED_UNIT(*)
SI_UNIT($,.STERADIAN.)
SOLID_ANGLE_UNIT()
);
#19069=SHAPE_DEFINITION_REPRESENTATION(#19139,#19327);
#19139=PRODUCT_DEFINITION_SHAPE('',$,#19398);
#19327=SHAPE_REPRESENTATION('',(#10579),#18994);
#19376=PRODUCT_DEFINITION_CONTEXT('part definition',#19588,'design');
#19398=PRODUCT_DEFINITION('2026-11-03-00-38-46-462','Pivot pedestal',#19468,
#19376);
#19468=PRODUCT_DEFINITION_FORMATION('',$,#19611);
#19588=APPLICATION_CONTEXT(
'Core Data for Automotive Mechanical Design Process');
#19589=PRODUCT_CONTEXT('part definition',#19588,'mechanical');
#19611=PRODUCT('2026-11-03-00-38-46-462','Pivot pedestal',
'Pivot pedestal',(#19589));
#19661=PRESENTATION_STYLE_ASSIGNMENT((#19667));
#19667=SURFACE_STYLE_USAGE(.BOTH.,#19673);
#19673=SURFACE_SIDE_STYLE('',(#19679));
#19679=SURFACE_STYLE_FILL_AREA(#19685);
#19685=FILL_AREA_STYLE('CAD Library Painted - Engineering blue',(#19691));
#19691=FILL_AREA_STYLE_COLOUR('CAD Library Painted - Engineering blue',
#19697);
#19697=COLOUR_RGB('CAD Library Painted - Engineering blue',0.12156862745098,
0.356862745098039,0.6);
ENDSEC;
END-ISO-10303-21;
